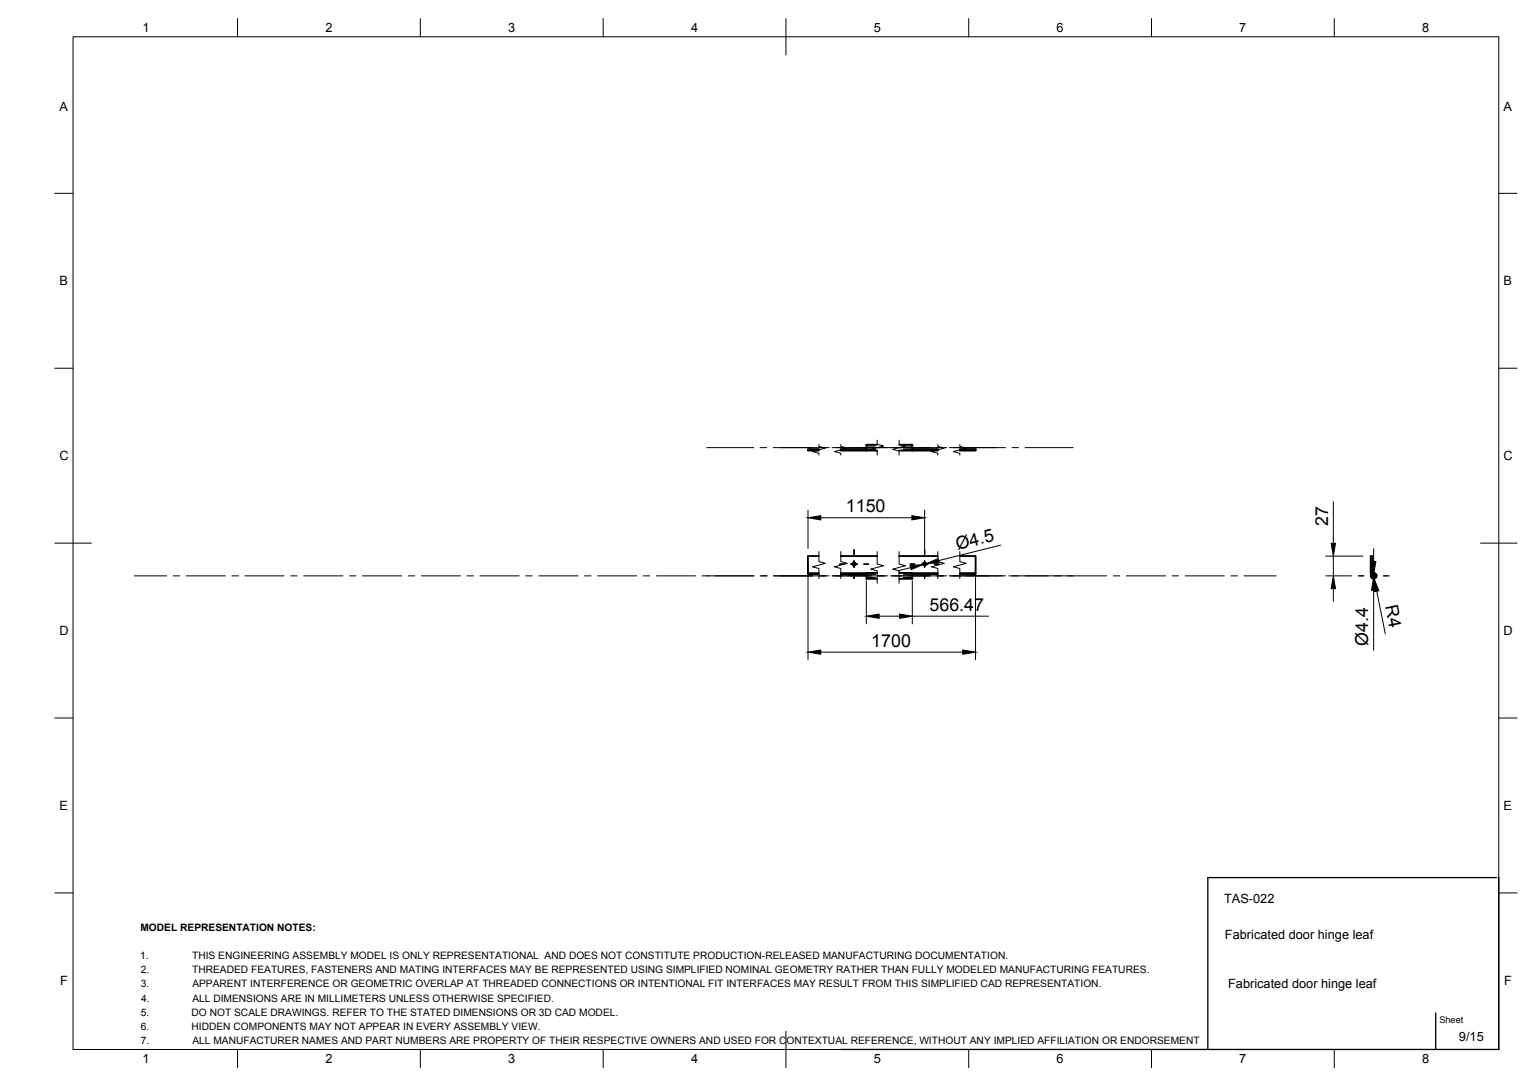
ISO-10303-21;
HEADER;
/* Generated by software containing ST-Developer
 * from STEP Tools, Inc. (www.steptools.com) 
 */

FILE_DESCRIPTION(
/* description */ (''),
/* implementation_level */ '2;1');

FILE_NAME(
/* name */ 'Fabricated door hinge leaf.step',
/* time_stamp */ '2026-11-15T21:02:08-08:00',
/* author */ (''),
/* organization */ (''),
/* preprocessor_version */ 'ST-DEVELOPER v20.2',
/* originating_system */ 'Autodesk Translation Framework v15.17.0.0',
/* authorisation */ '');

FILE_SCHEMA (('AUTOMOTIVE_DESIGN { 1 0 10303 214 3 1 1 }'));
ENDSEC;

DATA;
#10=MECHANICAL_DESIGN_GEOMETRIC_PRESENTATION_REPRESENTATION('',(#605),#31566);
#393=FACE_BOUND('',#954,.T.);
#394=FACE_BOUND('',#955,.T.);
#395=FACE_BOUND('',#961,.T.);
#396=FACE_BOUND('',#965,.T.);
#397=FACE_BOUND('',#967,.T.);
#398=FACE_BOUND('',#968,.T.);
#439=CIRCLE('',#5960,0.225);
#440=CIRCLE('',#5961,0.225);
#441=CIRCLE('',#5963,0.225);
#442=CIRCLE('',#5964,0.225);
#443=CIRCLE('',#5966,0.42);
#444=CIRCLE('',#5968,0.42);
#445=CIRCLE('',#5972,0.42);
#446=CIRCLE('',#5973,0.42);
#447=CIRCLE('',#5977,0.4);
#448=CIRCLE('',#5978,0.22);
#449=CIRCLE('',#5980,0.22);
#450=CIRCLE('',#5982,0.4);
#501=CYLINDRICAL_SURFACE('',#5959,0.225);
#502=CYLINDRICAL_SURFACE('',#5962,0.225);
#503=CYLINDRICAL_SURFACE('',#5967,0.42);
#504=CYLINDRICAL_SURFACE('',#5971,0.42);
#505=CYLINDRICAL_SURFACE('',#5979,0.22);
#506=CYLINDRICAL_SURFACE('',#5981,0.4);
#575=SHAPE_REPRESENTATION_RELATIONSHIP('SRR','None',#31639,#590);
#590=ADVANCED_BREP_SHAPE_REPRESENTATION('',(#620),#31554);
#605=STYLED_ITEM('',(#31720),#620);
#620=MANIFOLD_SOLID_BREP('Body1',#5718);
#668=FACE_OUTER_BOUND('',#949,.T.);
#669=FACE_OUTER_BOUND('',#950,.T.);
#670=FACE_OUTER_BOUND('',#951,.T.);
#671=FACE_OUTER_BOUND('',#952,.T.);
#672=FACE_OUTER_BOUND('',#953,.T.);
#673=FACE_OUTER_BOUND('',#956,.T.);
#674=FACE_OUTER_BOUND('',#957,.T.);
#675=FACE_OUTER_BOUND('',#958,.T.);
#676=FACE_OUTER_BOUND('',#959,.T.);
#677=FACE_OUTER_BOUND('',#960,.T.);
#678=FACE_OUTER_BOUND('',#962,.T.);
#679=FACE_OUTER_BOUND('',#963,.T.);
#680=FACE_OUTER_BOUND('',#964,.T.);
#681=FACE_OUTER_BOUND('',#966,.T.);
#682=FACE_OUTER_BOUND('',#969,.T.);
#683=FACE_OUTER_BOUND('',#970,.T.);
#949=EDGE_LOOP('',(#3819,#3820,#3821,#3822));
#950=EDGE_LOOP('',(#3823,#3824,#3825,#3826));
#951=EDGE_LOOP('',(#3827,#3828,#3829));
#952=EDGE_LOOP('',(#3830,#3831,#3832,#3833));
#953=EDGE_LOOP('',(#3834,#3835,#3836,#3837,#3838,#3839,#3840,#3841,#3842,
#3843,#3844,#3845));
#954=EDGE_LOOP('',(#3846));
#955=EDGE_LOOP('',(#3847));
#956=EDGE_LOOP('',(#3848,#3849,#3850,#3851,#3852,#3853,#3854,#3855,#3856,
#3857,#3858,#3859));
#957=EDGE_LOOP('',(#3860,#3861,#3862,#3863));
#958=EDGE_LOOP('',(#3864,#3865,#3866));
#959=EDGE_LOOP('',(#3867,#3868,#3869,#3870,#3871));
#960=EDGE_LOOP('',(#3872,#3873,#3874));
#961=EDGE_LOOP('',(#3875));
#962=EDGE_LOOP('',(#3876,#3877,#3878,#3879));
#963=EDGE_LOOP('',(#3880,#3881,#3882,#3883));
#964=EDGE_LOOP('',(#3884,#3885,#3886));
#965=EDGE_LOOP('',(#3887));
#966=EDGE_LOOP('',(#3888,#3889,#3890,#3891));
#967=EDGE_LOOP('',(#3892));
#968=EDGE_LOOP('',(#3893));
#969=EDGE_LOOP('',(#3894,#3895,#3896,#3897));
#970=EDGE_LOOP('',(#3898,#3899,#3900,#3901,#3902));
#1280=LINE('',#7766,#1787);
#1281=LINE('',#7772,#1788);
#1282=LINE('',#7777,#1789);
#1283=LINE('',#7780,#1790);
#1284=LINE('',#7783,#1791);
#1285=LINE('',#7786,#1792);
#1286=LINE('',#7789,#1793);
#1287=LINE('',#7791,#1794);
#1288=LINE('',#7793,#1795);
#1289=LINE('',#7795,#1796);
#1290=LINE('',#7797,#1797);
#1291=LINE('',#7799,#1798);
#1292=LINE('',#7801,#1799);
#1293=LINE('',#7803,#1800);
#1294=LINE('',#7805,#1801);
#1295=LINE('',#7806,#1802);
#1296=LINE('',#7809,#1803);
#1297=LINE('',#7811,#1804);
#1298=LINE('',#7813,#1805);
#1299=LINE('',#7815,#1806);
#1300=LINE('',#7816,#1807);
#1301=LINE('',#7818,#1808);
#1302=LINE('',#7820,#1809);
#1303=LINE('',#7821,#1810);
#1304=LINE('',#7828,#1811);
#1305=LINE('',#7829,#1812);
#1306=LINE('',#7837,#1813);
#1307=LINE('',#7843,#1814);
#1308=LINE('',#7844,#1815);
#1309=LINE('',#7846,#1816);
#1787=VECTOR('',#6486,0.225);
#1788=VECTOR('',#6493,0.225);
#1789=VECTOR('',#6498,1.);
#1790=VECTOR('',#6501,1.);
#1791=VECTOR('',#6504,1.);
#1792=VECTOR('',#6507,1.);
#1793=VECTOR('',#6510,1.);
#1794=VECTOR('',#6511,1.);
#1795=VECTOR('',#6512,1.);
#1796=VECTOR('',#6513,1.);
#1797=VECTOR('',#6514,1.);
#1798=VECTOR('',#6515,1.);
#1799=VECTOR('',#6516,1.);
#1800=VECTOR('',#6517,1.);
#1801=VECTOR('',#6518,1.);
#1802=VECTOR('',#6519,1.);
#1803=VECTOR('',#6522,1.);
#1804=VECTOR('',#6523,1.);
#1805=VECTOR('',#6524,1.);
#1806=VECTOR('',#6525,1.);
#1807=VECTOR('',#6526,1.);
#1808=VECTOR('',#6527,1.);
#1809=VECTOR('',#6528,1.);
#1810=VECTOR('',#6529,1.);
#1811=VECTOR('',#6540,1.);
#1812=VECTOR('',#6541,1.);
#1813=VECTOR('',#6552,0.22);
#1814=VECTOR('',#6561,1.);
#1815=VECTOR('',#6562,1.);
#1816=VECTOR('',#6565,1.);
#2284=VERTEX_POINT('',#7763);
#2285=VERTEX_POINT('',#7765);
#2286=VERTEX_POINT('',#7769);
#2287=VERTEX_POINT('',#7771);
#2288=VERTEX_POINT('',#7775);
#2289=VERTEX_POINT('',#7776);
#2290=VERTEX_POINT('',#7778);
#2291=VERTEX_POINT('',#7782);
#2292=VERTEX_POINT('',#7784);
#2293=VERTEX_POINT('',#7788);
#2294=VERTEX_POINT('',#7790);
#2295=VERTEX_POINT('',#7792);
#2296=VERTEX_POINT('',#7794);
#2297=VERTEX_POINT('',#7796);
#2298=VERTEX_POINT('',#7798);
#2299=VERTEX_POINT('',#7800);
#2300=VERTEX_POINT('',#7802);
#2301=VERTEX_POINT('',#7804);
#2302=VERTEX_POINT('',#7808);
#2303=VERTEX_POINT('',#7810);
#2304=VERTEX_POINT('',#7812);
#2305=VERTEX_POINT('',#7814);
#2306=VERTEX_POINT('',#7817);
#2307=VERTEX_POINT('',#7819);
#2308=VERTEX_POINT('',#7827);
#2309=VERTEX_POINT('',#7832);
#2310=VERTEX_POINT('',#7835);
#2311=VERTEX_POINT('',#7842);
#2905=EDGE_CURVE('',#2284,#2284,#439,.T.);
#2906=EDGE_CURVE('',#2284,#2285,#1280,.T.);
#2907=EDGE_CURVE('',#2285,#2285,#440,.T.);
#2908=EDGE_CURVE('',#2286,#2286,#441,.T.);
#2909=EDGE_CURVE('',#2286,#2287,#1281,.T.);
#2910=EDGE_CURVE('',#2287,#2287,#442,.T.);
#2911=EDGE_CURVE('',#2288,#2289,#1282,.T.);
#2912=EDGE_CURVE('',#2288,#2290,#443,.T.);
#2913=EDGE_CURVE('',#2289,#2290,#1283,.T.);
#2914=EDGE_CURVE('',#2291,#2288,#1284,.T.);
#2915=EDGE_CURVE('',#2292,#2291,#444,.T.);
#2916=EDGE_CURVE('',#2290,#2292,#1285,.T.);
#2917=EDGE_CURVE('',#2293,#2289,#1286,.T.);
#2918=EDGE_CURVE('',#2293,#2294,#1287,.T.);
#2919=EDGE_CURVE('',#2294,#2295,#1288,.T.);
#2920=EDGE_CURVE('',#2295,#2296,#1289,.T.);
#2921=EDGE_CURVE('',#2297,#2296,#1290,.T.);
#2922=EDGE_CURVE('',#2297,#2298,#1291,.T.);
#2923=EDGE_CURVE('',#2298,#2299,#1292,.T.);
#2924=EDGE_CURVE('',#2299,#2300,#1293,.T.);
#2925=EDGE_CURVE('',#2300,#2301,#1294,.T.);
#2926=EDGE_CURVE('',#2291,#2301,#1295,.T.);
#2927=EDGE_CURVE('',#2302,#2292,#1296,.T.);
#2928=EDGE_CURVE('',#2303,#2302,#1297,.T.);
#2929=EDGE_CURVE('',#2303,#2304,#1298,.T.);
#2930=EDGE_CURVE('',#2304,#2305,#1299,.T.);
#2931=EDGE_CURVE('',#2305,#2297,#1300,.T.);
#2932=EDGE_CURVE('',#2296,#2306,#1301,.T.);
#2933=EDGE_CURVE('',#2306,#2307,#1302,.T.);
#2934=EDGE_CURVE('',#2307,#2293,#1303,.T.);
#2935=EDGE_CURVE('',#2298,#2305,#445,.T.);
#2936=EDGE_CURVE('',#2299,#2304,#446,.T.);
#2937=EDGE_CURVE('',#2308,#2303,#1304,.T.);
#2938=EDGE_CURVE('',#2300,#2308,#1305,.T.);
#2939=EDGE_CURVE('',#2307,#2294,#447,.T.);
#2940=EDGE_CURVE('',#2309,#2309,#448,.T.);
#2941=EDGE_CURVE('',#2310,#2310,#449,.T.);
#2942=EDGE_CURVE('',#2310,#2309,#1306,.T.);
#2943=EDGE_CURVE('',#2306,#2295,#450,.T.);
#2944=EDGE_CURVE('',#2311,#2302,#1307,.T.);
#2945=EDGE_CURVE('',#2308,#2311,#1308,.T.);
#2946=EDGE_CURVE('',#2301,#2311,#1309,.T.);
#3819=ORIENTED_EDGE('',*,*,#2905,.F.);
#3820=ORIENTED_EDGE('',*,*,#2906,.T.);
#3821=ORIENTED_EDGE('',*,*,#2907,.F.);
#3822=ORIENTED_EDGE('',*,*,#2906,.F.);
#3823=ORIENTED_EDGE('',*,*,#2908,.F.);
#3824=ORIENTED_EDGE('',*,*,#2909,.T.);
#3825=ORIENTED_EDGE('',*,*,#2910,.F.);
#3826=ORIENTED_EDGE('',*,*,#2909,.F.);
#3827=ORIENTED_EDGE('',*,*,#2911,.F.);
#3828=ORIENTED_EDGE('',*,*,#2912,.T.);
#3829=ORIENTED_EDGE('',*,*,#2913,.F.);
#3830=ORIENTED_EDGE('',*,*,#2914,.F.);
#3831=ORIENTED_EDGE('',*,*,#2915,.F.);
#3832=ORIENTED_EDGE('',*,*,#2916,.F.);
#3833=ORIENTED_EDGE('',*,*,#2912,.F.);
#3834=ORIENTED_EDGE('',*,*,#2914,.T.);
#3835=ORIENTED_EDGE('',*,*,#2911,.T.);
#3836=ORIENTED_EDGE('',*,*,#2917,.F.);
#3837=ORIENTED_EDGE('',*,*,#2918,.T.);
#3838=ORIENTED_EDGE('',*,*,#2919,.T.);
#3839=ORIENTED_EDGE('',*,*,#2920,.T.);
#3840=ORIENTED_EDGE('',*,*,#2921,.F.);
#3841=ORIENTED_EDGE('',*,*,#2922,.T.);
#3842=ORIENTED_EDGE('',*,*,#2923,.T.);
#3843=ORIENTED_EDGE('',*,*,#2924,.T.);
#3844=ORIENTED_EDGE('',*,*,#2925,.T.);
#3845=ORIENTED_EDGE('',*,*,#2926,.F.);
#3846=ORIENTED_EDGE('',*,*,#2907,.T.);
#3847=ORIENTED_EDGE('',*,*,#2910,.T.);
#3848=ORIENTED_EDGE('',*,*,#2913,.T.);
#3849=ORIENTED_EDGE('',*,*,#2916,.T.);
#3850=ORIENTED_EDGE('',*,*,#2927,.F.);
#3851=ORIENTED_EDGE('',*,*,#2928,.F.);
#3852=ORIENTED_EDGE('',*,*,#2929,.T.);
#3853=ORIENTED_EDGE('',*,*,#2930,.T.);
#3854=ORIENTED_EDGE('',*,*,#2931,.T.);
#3855=ORIENTED_EDGE('',*,*,#2921,.T.);
#3856=ORIENTED_EDGE('',*,*,#2932,.T.);
#3857=ORIENTED_EDGE('',*,*,#2933,.T.);
#3858=ORIENTED_EDGE('',*,*,#2934,.T.);
#3859=ORIENTED_EDGE('',*,*,#2917,.T.);
#3860=ORIENTED_EDGE('',*,*,#2923,.F.);
#3861=ORIENTED_EDGE('',*,*,#2935,.T.);
#3862=ORIENTED_EDGE('',*,*,#2930,.F.);
#3863=ORIENTED_EDGE('',*,*,#2936,.F.);
#3864=ORIENTED_EDGE('',*,*,#2922,.F.);
#3865=ORIENTED_EDGE('',*,*,#2931,.F.);
#3866=ORIENTED_EDGE('',*,*,#2935,.F.);
#3867=ORIENTED_EDGE('',*,*,#2936,.T.);
#3868=ORIENTED_EDGE('',*,*,#2929,.F.);
#3869=ORIENTED_EDGE('',*,*,#2937,.F.);
#3870=ORIENTED_EDGE('',*,*,#2938,.F.);
#3871=ORIENTED_EDGE('',*,*,#2924,.F.);
#3872=ORIENTED_EDGE('',*,*,#2918,.F.);
#3873=ORIENTED_EDGE('',*,*,#2934,.F.);
#3874=ORIENTED_EDGE('',*,*,#2939,.T.);
#3875=ORIENTED_EDGE('',*,*,#2940,.T.);
#3876=ORIENTED_EDGE('',*,*,#2941,.T.);
#3877=ORIENTED_EDGE('',*,*,#2942,.T.);
#3878=ORIENTED_EDGE('',*,*,#2940,.F.);
#3879=ORIENTED_EDGE('',*,*,#2942,.F.);
#3880=ORIENTED_EDGE('',*,*,#2919,.F.);
#3881=ORIENTED_EDGE('',*,*,#2939,.F.);
#3882=ORIENTED_EDGE('',*,*,#2933,.F.);
#3883=ORIENTED_EDGE('',*,*,#2943,.T.);
#3884=ORIENTED_EDGE('',*,*,#2920,.F.);
#3885=ORIENTED_EDGE('',*,*,#2943,.F.);
#3886=ORIENTED_EDGE('',*,*,#2932,.F.);
#3887=ORIENTED_EDGE('',*,*,#2941,.F.);
#3888=ORIENTED_EDGE('',*,*,#2937,.T.);
#3889=ORIENTED_EDGE('',*,*,#2928,.T.);
#3890=ORIENTED_EDGE('',*,*,#2944,.F.);
#3891=ORIENTED_EDGE('',*,*,#2945,.F.);
#3892=ORIENTED_EDGE('',*,*,#2905,.T.);
#3893=ORIENTED_EDGE('',*,*,#2908,.T.);
#3894=ORIENTED_EDGE('',*,*,#2938,.T.);
#3895=ORIENTED_EDGE('',*,*,#2945,.T.);
#3896=ORIENTED_EDGE('',*,*,#2946,.F.);
#3897=ORIENTED_EDGE('',*,*,#2925,.F.);
#3898=ORIENTED_EDGE('',*,*,#2915,.T.);
#3899=ORIENTED_EDGE('',*,*,#2926,.T.);
#3900=ORIENTED_EDGE('',*,*,#2946,.T.);
#3901=ORIENTED_EDGE('',*,*,#2944,.T.);
#3902=ORIENTED_EDGE('',*,*,#2927,.T.);
#5288=PLANE('',#5965);
#5289=PLANE('',#5969);
#5290=PLANE('',#5970);
#5291=PLANE('',#5974);
#5292=PLANE('',#5975);
#5293=PLANE('',#5976);
#5294=PLANE('',#5983);
#5295=PLANE('',#5984);
#5296=PLANE('',#5985);
#5297=PLANE('',#5986);
#5482=ADVANCED_FACE('',(#668),#501,.F.);
#5483=ADVANCED_FACE('',(#669),#502,.F.);
#5484=ADVANCED_FACE('',(#670),#5288,.T.);
#5485=ADVANCED_FACE('',(#671),#503,.F.);
#5486=ADVANCED_FACE('',(#672,#393,#394),#5289,.T.);
#5487=ADVANCED_FACE('',(#673),#5290,.T.);
#5488=ADVANCED_FACE('',(#674),#504,.F.);
#5489=ADVANCED_FACE('',(#675),#5291,.F.);
#5490=ADVANCED_FACE('',(#676),#5292,.F.);
#5491=ADVANCED_FACE('',(#677,#395),#5293,.T.);
#5492=ADVANCED_FACE('',(#678),#505,.F.);
#5493=ADVANCED_FACE('',(#679),#506,.T.);
#5494=ADVANCED_FACE('',(#680,#396),#5294,.F.);
#5495=ADVANCED_FACE('',(#681,#397,#398),#5295,.T.);
#5496=ADVANCED_FACE('',(#682),#5296,.T.);
#5497=ADVANCED_FACE('',(#683),#5297,.T.);
#5718=CLOSED_SHELL('',(#5482,#5483,#5484,#5485,#5486,#5487,#5488,#5489,
#5490,#5491,#5492,#5493,#5494,#5495,#5496,#5497));
#5958=AXIS2_PLACEMENT_3D('',#7761,#6480,#6481);
#5959=AXIS2_PLACEMENT_3D('',#7762,#6482,#6483);
#5960=AXIS2_PLACEMENT_3D('',#7764,#6484,#6485);
#5961=AXIS2_PLACEMENT_3D('',#7767,#6487,#6488);
#5962=AXIS2_PLACEMENT_3D('',#7768,#6489,#6490);
#5963=AXIS2_PLACEMENT_3D('',#7770,#6491,#6492);
#5964=AXIS2_PLACEMENT_3D('',#7773,#6494,#6495);
#5965=AXIS2_PLACEMENT_3D('',#7774,#6496,#6497);
#5966=AXIS2_PLACEMENT_3D('',#7779,#6499,#6500);
#5967=AXIS2_PLACEMENT_3D('',#7781,#6502,#6503);
#5968=AXIS2_PLACEMENT_3D('',#7785,#6505,#6506);
#5969=AXIS2_PLACEMENT_3D('',#7787,#6508,#6509);
#5970=AXIS2_PLACEMENT_3D('',#7807,#6520,#6521);
#5971=AXIS2_PLACEMENT_3D('',#7822,#6530,#6531);
#5972=AXIS2_PLACEMENT_3D('',#7823,#6532,#6533);
#5973=AXIS2_PLACEMENT_3D('',#7824,#6534,#6535);
#5974=AXIS2_PLACEMENT_3D('',#7825,#6536,#6537);
#5975=AXIS2_PLACEMENT_3D('',#7826,#6538,#6539);
#5976=AXIS2_PLACEMENT_3D('',#7830,#6542,#6543);
#5977=AXIS2_PLACEMENT_3D('',#7831,#6544,#6545);
#5978=AXIS2_PLACEMENT_3D('',#7833,#6546,#6547);
#5979=AXIS2_PLACEMENT_3D('',#7834,#6548,#6549);
#5980=AXIS2_PLACEMENT_3D('',#7836,#6550,#6551);
#5981=AXIS2_PLACEMENT_3D('',#7838,#6553,#6554);
#5982=AXIS2_PLACEMENT_3D('',#7839,#6555,#6556);
#5983=AXIS2_PLACEMENT_3D('',#7840,#6557,#6558);
#5984=AXIS2_PLACEMENT_3D('',#7841,#6559,#6560);
#5985=AXIS2_PLACEMENT_3D('',#7845,#6563,#6564);
#5986=AXIS2_PLACEMENT_3D('',#7847,#6566,#6567);
#6480=DIRECTION('axis',(0.,0.,1.));
#6481=DIRECTION('refdir',(1.,0.,0.));
#6482=DIRECTION('center_axis',(0.,-1.,0.));
#6483=DIRECTION('ref_axis',(1.,0.,0.));
#6484=DIRECTION('center_axis',(0.,-1.,0.));
#6485=DIRECTION('ref_axis',(1.,0.,0.));
#6486=DIRECTION('',(0.,-1.,0.));
#6487=DIRECTION('center_axis',(0.,1.,0.));
#6488=DIRECTION('ref_axis',(1.,0.,0.));
#6489=DIRECTION('center_axis',(0.,-1.,0.));
#6490=DIRECTION('ref_axis',(1.,0.,0.));
#6491=DIRECTION('center_axis',(0.,-1.,0.));
#6492=DIRECTION('ref_axis',(1.,0.,0.));
#6493=DIRECTION('',(0.,-1.,0.));
#6494=DIRECTION('center_axis',(0.,1.,0.));
#6495=DIRECTION('ref_axis',(1.,0.,0.));
#6496=DIRECTION('center_axis',(0.,0.,1.));
#6497=DIRECTION('ref_axis',(1.,0.,0.));
#6498=DIRECTION('',(-1.,0.,0.));
#6499=DIRECTION('center_axis',(0.,0.,1.));
#6500=DIRECTION('ref_axis',(1.,0.,0.));
#6501=DIRECTION('',(0.,1.,0.));
#6502=DIRECTION('center_axis',(0.,0.,1.));
#6503=DIRECTION('ref_axis',(1.,0.,0.));
#6504=DIRECTION('',(0.,0.,-1.));
#6505=DIRECTION('center_axis',(0.,0.,-1.));
#6506=DIRECTION('ref_axis',(1.,0.,0.));
#6507=DIRECTION('',(0.,0.,1.));
#6508=DIRECTION('center_axis',(0.,-1.,0.));
#6509=DIRECTION('ref_axis',(1.,0.,0.));
#6510=DIRECTION('',(0.,0.,1.));
#6511=DIRECTION('',(1.,0.,0.));
#6512=DIRECTION('',(0.,0.,-1.));
#6513=DIRECTION('',(-1.,0.,0.));
#6514=DIRECTION('',(0.,0.,1.));
#6515=DIRECTION('',(1.,0.,0.));
#6516=DIRECTION('',(0.,0.,-1.));
#6517=DIRECTION('',(1.,0.,0.));
#6518=DIRECTION('',(0.,0.,1.));
#6519=DIRECTION('',(1.,0.,0.));
#6520=DIRECTION('center_axis',(-1.,0.,0.));
#6521=DIRECTION('ref_axis',(0.,-1.,0.));
#6522=DIRECTION('',(0.,-1.,0.));
#6523=DIRECTION('',(0.,0.,1.));
#6524=DIRECTION('',(0.,-1.,0.));
#6525=DIRECTION('',(0.,0.,1.));
#6526=DIRECTION('',(0.,-1.,0.));
#6527=DIRECTION('',(0.,1.,0.));
#6528=DIRECTION('',(0.,0.,1.));
#6529=DIRECTION('',(0.,-1.,0.));
#6530=DIRECTION('center_axis',(0.,0.,1.));
#6531=DIRECTION('ref_axis',(1.,0.,0.));
#6532=DIRECTION('center_axis',(0.,0.,1.));
#6533=DIRECTION('ref_axis',(1.,0.,0.));
#6534=DIRECTION('center_axis',(0.,0.,1.));
#6535=DIRECTION('ref_axis',(1.,0.,0.));
#6536=DIRECTION('center_axis',(0.,0.,1.));
#6537=DIRECTION('ref_axis',(1.,0.,0.));
#6538=DIRECTION('center_axis',(0.,0.,1.));
#6539=DIRECTION('ref_axis',(1.,0.,0.));
#6540=DIRECTION('',(-1.,0.,0.));
#6541=DIRECTION('',(0.,1.,0.));
#6542=DIRECTION('center_axis',(0.,0.,1.));
#6543=DIRECTION('ref_axis',(1.,0.,0.));
#6544=DIRECTION('center_axis',(0.,0.,1.));
#6545=DIRECTION('ref_axis',(1.,0.,0.));
#6546=DIRECTION('center_axis',(0.,0.,-1.));
#6547=DIRECTION('ref_axis',(1.,0.,0.));
#6548=DIRECTION('center_axis',(0.,0.,1.));
#6549=DIRECTION('ref_axis',(1.,0.,0.));
#6550=DIRECTION('center_axis',(0.,0.,-1.));
#6551=DIRECTION('ref_axis',(1.,0.,0.));
#6552=DIRECTION('',(0.,0.,1.));
#6553=DIRECTION('center_axis',(0.,0.,1.));
#6554=DIRECTION('ref_axis',(-0.758601839724033,-0.651554486414845,0.));
#6555=DIRECTION('center_axis',(0.,0.,1.));
#6556=DIRECTION('ref_axis',(1.,0.,0.));
#6557=DIRECTION('center_axis',(0.,0.,1.));
#6558=DIRECTION('ref_axis',(1.,0.,0.));
#6559=DIRECTION('center_axis',(0.,1.,0.));
#6560=DIRECTION('ref_axis',(-1.,0.,0.));
#6561=DIRECTION('',(-1.,0.,0.));
#6562=DIRECTION('',(0.,0.,1.));
#6563=DIRECTION('center_axis',(1.,0.,0.));
#6564=DIRECTION('ref_axis',(0.,1.,0.));
#6565=DIRECTION('',(0.,1.,0.));
#6566=DIRECTION('center_axis',(0.,0.,1.));
#6567=DIRECTION('ref_axis',(1.,0.,0.));
#7761=CARTESIAN_POINT('',(0.,0.,0.));
#7762=CARTESIAN_POINT('Origin',(1.6,0.4,55.));
#7763=CARTESIAN_POINT('',(1.375,0.4,55.));
#7764=CARTESIAN_POINT('Origin',(1.6,0.4,55.));
#7765=CARTESIAN_POINT('',(1.375,0.2,55.));
#7766=CARTESIAN_POINT('',(1.375,0.4,55.));
#7767=CARTESIAN_POINT('Origin',(1.6,0.2,55.));
#7768=CARTESIAN_POINT('Origin',(1.6,0.4,115.));
#7769=CARTESIAN_POINT('',(1.375,0.4,115.));
#7770=CARTESIAN_POINT('Origin',(1.6,0.4,115.));
#7771=CARTESIAN_POINT('',(1.375,0.2,115.));
#7772=CARTESIAN_POINT('',(1.375,0.4,115.));
#7773=CARTESIAN_POINT('Origin',(1.6,0.2,115.));
#7774=CARTESIAN_POINT('Origin',(0.,0.,113.323333333333));
#7775=CARTESIAN_POINT('',(0.369323706252388,0.2,113.323333333333));
#7776=CARTESIAN_POINT('',(0.25,0.2,113.323333333333));
#7777=CARTESIAN_POINT('',(0.125,0.2,113.323333333333));
#7778=CARTESIAN_POINT('',(0.25,0.337490740613724,113.323333333333));
#7779=CARTESIAN_POINT('Origin',(0.,0.,113.323333333333));
#7780=CARTESIAN_POINT('',(0.25,0.2,113.323333333333));
#7781=CARTESIAN_POINT('Origin',(0.,0.,113.323333333333));
#7782=CARTESIAN_POINT('',(0.369323706252388,0.2,170.));
#7783=CARTESIAN_POINT('',(0.369323706252388,0.2,113.323333333333));
#7784=CARTESIAN_POINT('',(0.25,0.337490740613724,170.));
#7785=CARTESIAN_POINT('Origin',(0.,0.,170.));
#7786=CARTESIAN_POINT('',(0.25,0.337490740613724,113.323333333333));
#7787=CARTESIAN_POINT('Origin',(0.25,0.2,0.));
#7788=CARTESIAN_POINT('',(0.25,0.2,113.313333333333));
#7789=CARTESIAN_POINT('',(0.25,0.2,0.));
#7790=CARTESIAN_POINT('',(0.346410161513776,0.2,113.313333333333));
#7791=CARTESIAN_POINT('',(0.125,0.2,113.313333333333));
#7792=CARTESIAN_POINT('',(0.346410161513776,0.2,56.6866666666667));
#7793=CARTESIAN_POINT('',(0.346410161513776,0.2,56.6866666666667));
#7794=CARTESIAN_POINT('',(0.25,0.2,56.6866666666667));
#7795=CARTESIAN_POINT('',(0.125,0.2,56.6866666666667));
#7796=CARTESIAN_POINT('',(0.25,0.2,56.6766666666667));
#7797=CARTESIAN_POINT('',(0.25,0.2,0.));
#7798=CARTESIAN_POINT('',(0.369323706252388,0.2,56.6766666666667));
#7799=CARTESIAN_POINT('',(0.125,0.2,56.6766666666667));
#7800=CARTESIAN_POINT('',(0.369323706252388,0.2,0.));
#7801=CARTESIAN_POINT('',(0.369323706252388,0.2,0.));
#7802=CARTESIAN_POINT('',(2.7,0.2,0.));
#7803=CARTESIAN_POINT('',(0.25,0.2,0.));
#7804=CARTESIAN_POINT('',(2.7,0.2,170.));
#7805=CARTESIAN_POINT('',(2.7,0.2,0.));
#7806=CARTESIAN_POINT('',(0.25,0.2,170.));
#7807=CARTESIAN_POINT('Origin',(0.25,0.4,0.));
#7808=CARTESIAN_POINT('',(0.25,0.4,170.));
#7809=CARTESIAN_POINT('',(0.25,0.4,170.));
#7810=CARTESIAN_POINT('',(0.25,0.4,0.));
#7811=CARTESIAN_POINT('',(0.25,0.4,0.));
#7812=CARTESIAN_POINT('',(0.25,0.337490740613724,0.));
#7813=CARTESIAN_POINT('',(0.25,0.4,0.));
#7814=CARTESIAN_POINT('',(0.25,0.337490740613724,56.6766666666667));
#7815=CARTESIAN_POINT('',(0.25,0.337490740613724,0.));
#7816=CARTESIAN_POINT('',(0.25,0.2,56.6766666666667));
#7817=CARTESIAN_POINT('',(0.25,0.31224989991992,56.6866666666667));
#7818=CARTESIAN_POINT('',(0.25,0.2,56.6866666666667));
#7819=CARTESIAN_POINT('',(0.25,0.31224989991992,113.313333333333));
#7820=CARTESIAN_POINT('',(0.25,0.31224989991992,56.6866666666667));
#7821=CARTESIAN_POINT('',(0.25,0.2,113.313333333333));
#7822=CARTESIAN_POINT('Origin',(0.,0.,0.));
#7823=CARTESIAN_POINT('Origin',(0.,0.,56.6766666666667));
#7824=CARTESIAN_POINT('Origin',(0.,0.,0.));
#7825=CARTESIAN_POINT('Origin',(0.,0.,56.6766666666667));
#7826=CARTESIAN_POINT('Origin',(1.475,0.3,0.));
#7827=CARTESIAN_POINT('',(2.7,0.4,0.));
#7828=CARTESIAN_POINT('',(2.7,0.4,0.));
#7829=CARTESIAN_POINT('',(2.7,0.2,0.));
#7830=CARTESIAN_POINT('Origin',(0.,0.,113.313333333333));
#7831=CARTESIAN_POINT('Origin',(0.,0.,113.313333333333));
#7832=CARTESIAN_POINT('',(-0.22,-2.69422295812418E-17,113.313333333333));
#7833=CARTESIAN_POINT('Origin',(0.,0.,113.313333333333));
#7834=CARTESIAN_POINT('Origin',(0.,0.,56.6866666666667));
#7835=CARTESIAN_POINT('',(-0.22,-2.69422295812418E-17,56.6866666666667));
#7836=CARTESIAN_POINT('Origin',(0.,0.,56.6866666666667));
#7837=CARTESIAN_POINT('',(-0.22,-2.69422295812418E-17,56.6866666666667));
#7838=CARTESIAN_POINT('Origin',(0.,0.,56.6866666666667));
#7839=CARTESIAN_POINT('Origin',(0.,0.,56.6866666666667));
#7840=CARTESIAN_POINT('Origin',(0.,0.,56.6866666666667));
#7841=CARTESIAN_POINT('Origin',(2.7,0.4,0.));
#7842=CARTESIAN_POINT('',(2.7,0.4,170.));
#7843=CARTESIAN_POINT('',(2.7,0.4,170.));
#7844=CARTESIAN_POINT('',(2.7,0.4,0.));
#7845=CARTESIAN_POINT('Origin',(2.7,0.2,0.));
#7846=CARTESIAN_POINT('',(2.7,0.2,170.));
#7847=CARTESIAN_POINT('Origin',(1.475,0.3,170.));
#31537=UNCERTAINTY_MEASURE_WITH_UNIT(LENGTH_MEASURE(0.001),#31567,
'DISTANCE_ACCURACY_VALUE',
'Maximum model space distance between geometric entities at asserted c
onnectivities');
#31549=UNCERTAINTY_MEASURE_WITH_UNIT(LENGTH_MEASURE(0.001),#31567,
'DISTANCE_ACCURACY_VALUE',
'Maximum model space distance between geometric entities at asserted c
onnectivities');
#31554=(
GEOMETRIC_REPRESENTATION_CONTEXT(3)
GLOBAL_UNCERTAINTY_ASSIGNED_CONTEXT((#31537))
GLOBAL_UNIT_ASSIGNED_CONTEXT((#31567,#31569,#31570))
REPRESENTATION_CONTEXT('','3D')
);
#31566=(
GEOMETRIC_REPRESENTATION_CONTEXT(3)
GLOBAL_UNCERTAINTY_ASSIGNED_CONTEXT((#31549))
GLOBAL_UNIT_ASSIGNED_CONTEXT((#31567,#31569,#31570))
REPRESENTATION_CONTEXT('','3D')
);
#31567=(
LENGTH_UNIT()
NAMED_UNIT(*)
SI_UNIT(.CENTI.,.METRE.)
);
#31569=(
NAMED_UNIT(*)
PLANE_ANGLE_UNIT()
SI_UNIT($,.RADIAN.)
);
#31570=(
NAMED_UNIT(*)
SI_UNIT($,.STERADIAN.)
SOLID_ANGLE_UNIT()
);
#31575=SHAPE_DEFINITION_REPRESENTATION(#31591,#31639);
#31591=PRODUCT_DEFINITION_SHAPE('',$,#31656);
#31639=SHAPE_REPRESENTATION('',(#5958),#31554);
#31651=PRODUCT_DEFINITION_CONTEXT('part definition',#31701,'design');
#31656=PRODUCT_DEFINITION('Fabricated door hinge leaf',
'Fabricated door hinge leaf',#31672,#31651);
#31672=PRODUCT_DEFINITION_FORMATION('',$,#31707);
#31701=APPLICATION_CONTEXT(
'Core Data for Automotive Mechanical Design Process');
#31702=PRODUCT_CONTEXT('part definition',#31701,'mechanical');
#31707=PRODUCT('Fabricated door hinge leaf',
'Fabricated door hinge leaf',$,(#31702));
#31720=PRESENTATION_STYLE_ASSIGNMENT((#31727));
#31727=SURFACE_STYLE_USAGE(.BOTH.,#31734);
#31734=SURFACE_SIDE_STYLE('',(#31741));
#31741=SURFACE_STYLE_FILL_AREA(#31748);
#31748=FILL_AREA_STYLE('Opaque(155,165,179)',(#31755));
#31755=FILL_AREA_STYLE_COLOUR('Opaque(155,165,179)',#31762);
#31762=COLOUR_RGB('Opaque(155,165,179)',0.607843137254902,0.647058823529412,
0.701960784313725);
ENDSEC;
END-ISO-10303-21;
